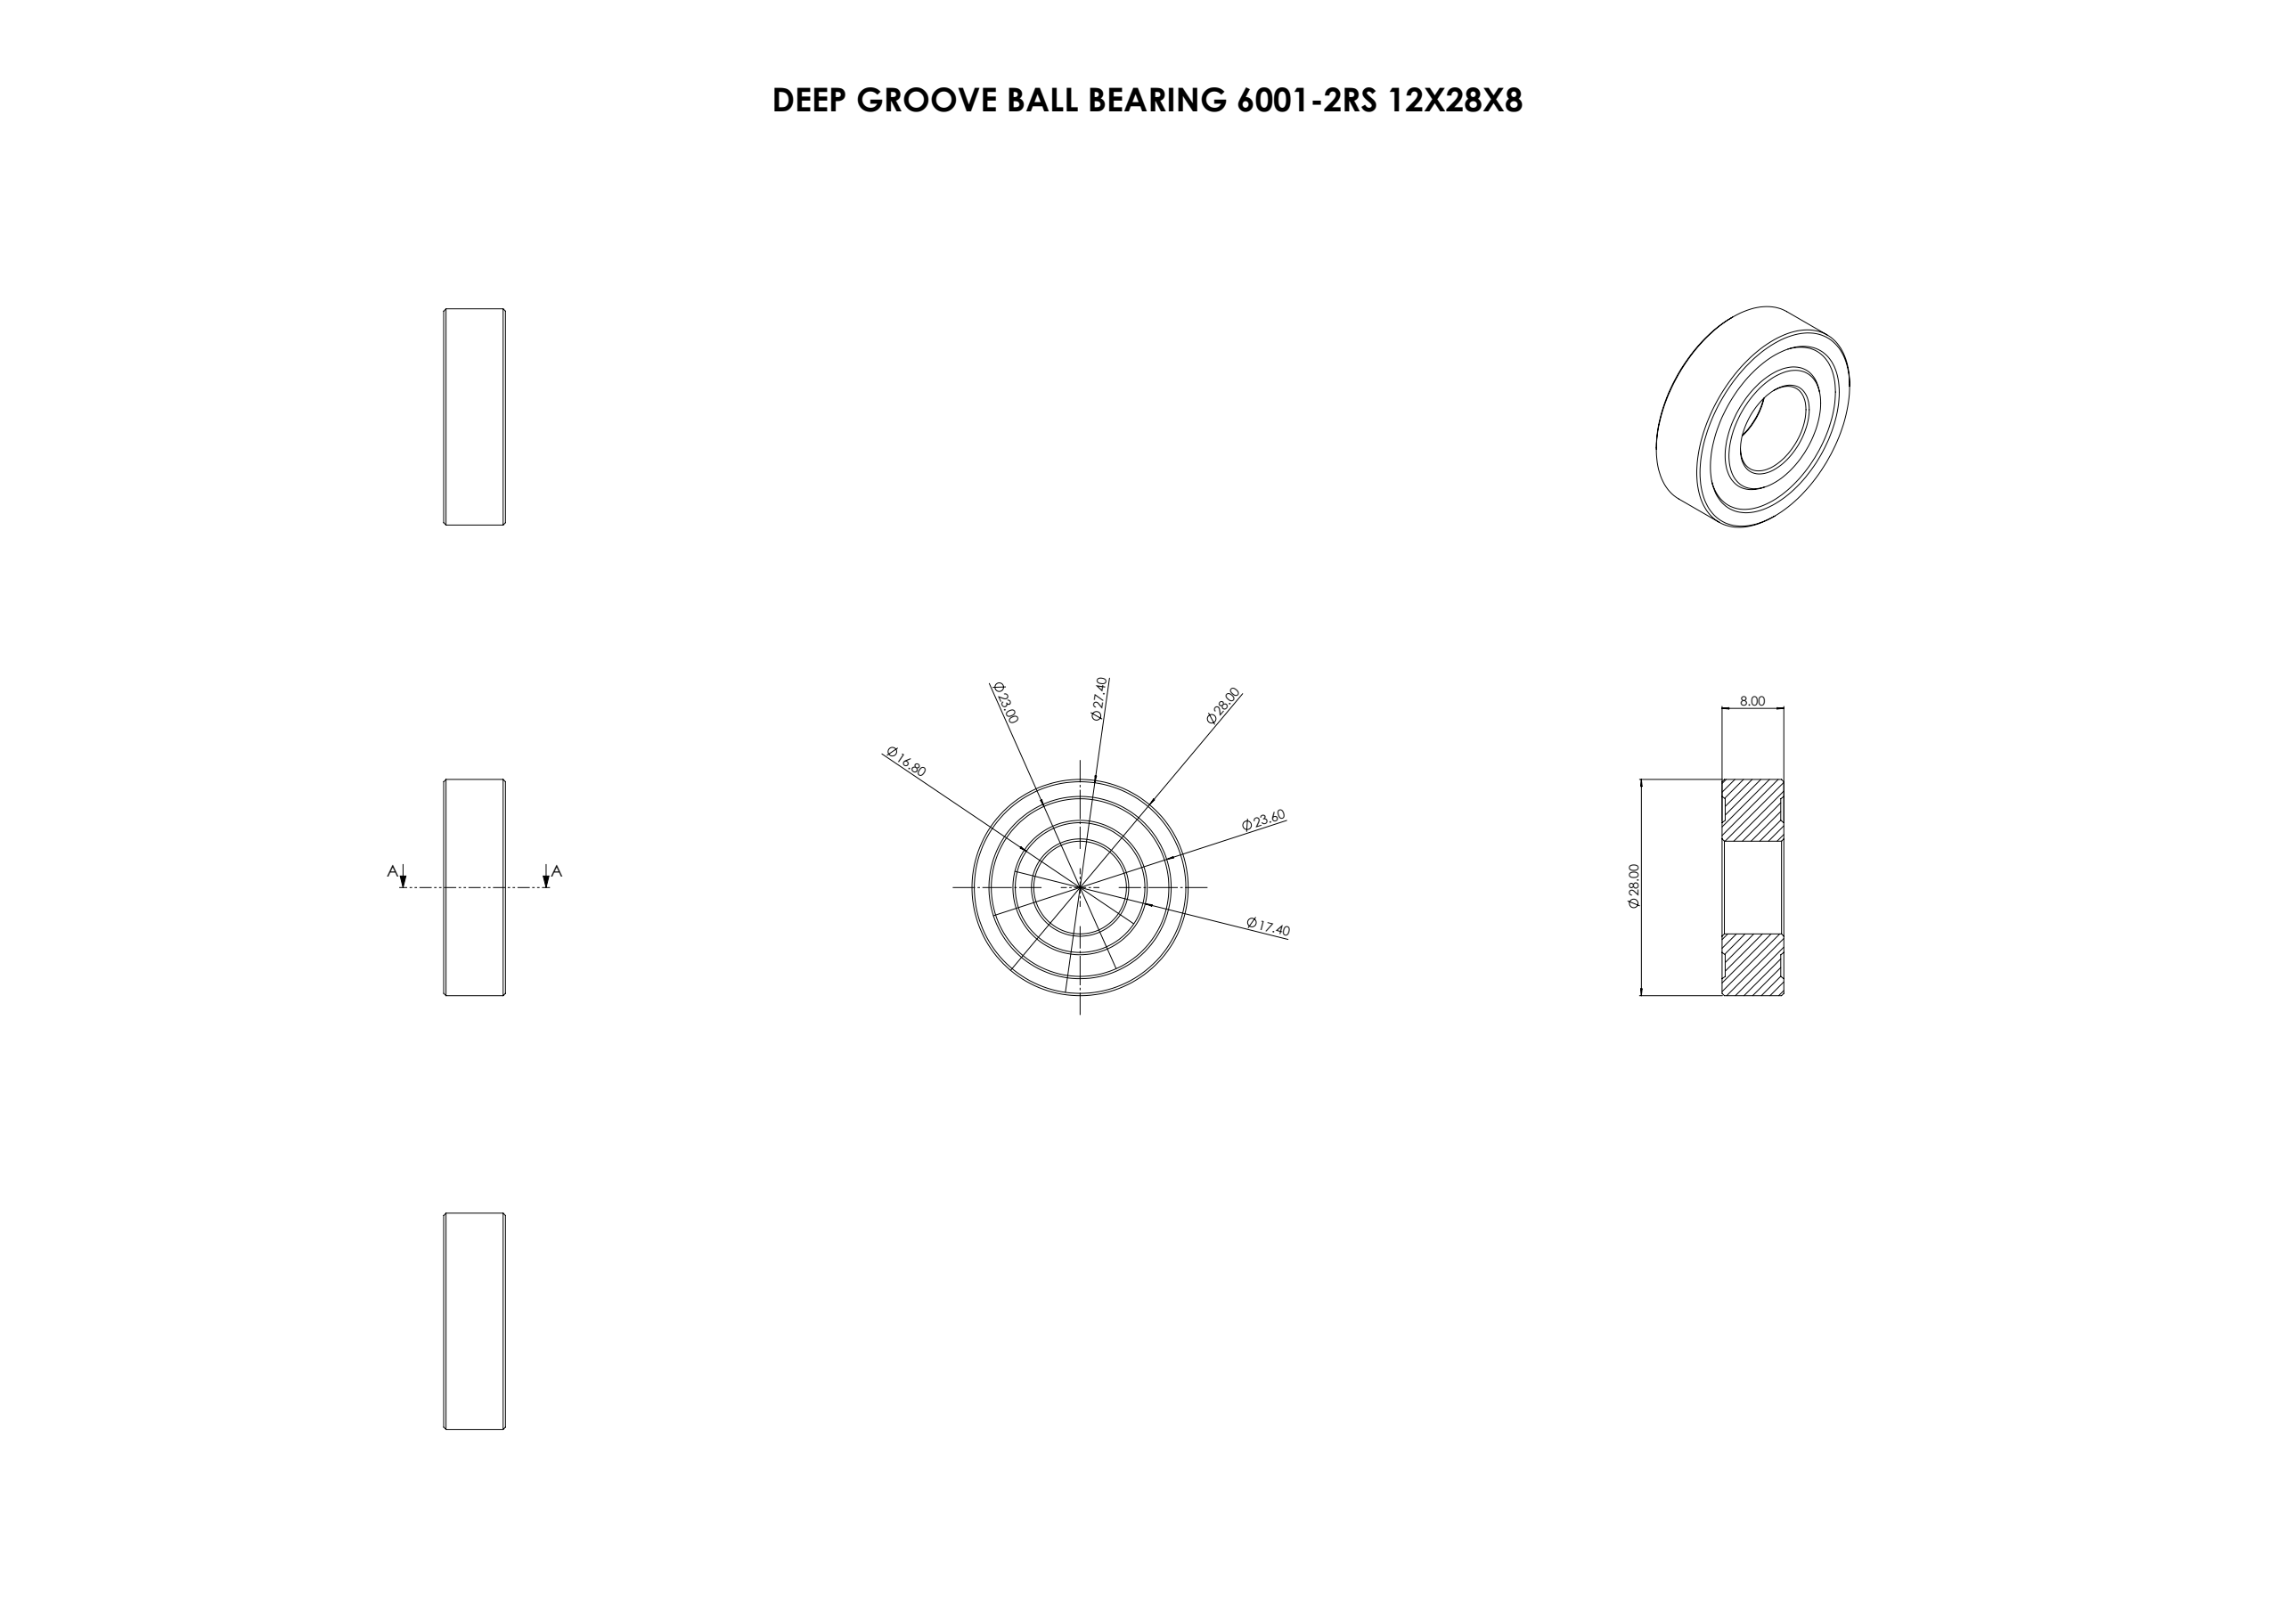
ISO-10303-21;
HEADER;
/* Generated by software containing ST-Developer
 * from STEP Tools, Inc. (www.steptools.com) 
 */

FILE_DESCRIPTION(
/* description */ (''),
/* implementation_level */ '2;1');

FILE_NAME(
/* name */ '07_Deep_Groove_Ball_Bearing_6001-2RS_12x28x8.step',
/* time_stamp */ '2026-10-11T09:12:28-07:00',
/* author */ (''),
/* organization */ (''),
/* preprocessor_version */ 'ST-DEVELOPER v20.2',
/* originating_system */ 'Autodesk Translation Framework v15.15.0.0',
/* authorisation */ '');

FILE_SCHEMA (('AUTOMOTIVE_DESIGN { 1 0 10303 214 3 1 1 }'));
ENDSEC;

DATA;
#10=MECHANICAL_DESIGN_GEOMETRIC_PRESENTATION_REPRESENTATION('',(#653),#23254);
#633=SHAPE_REPRESENTATION_RELATIONSHIP('SRR','None',#23306,#643);
#643=ADVANCED_BREP_SHAPE_REPRESENTATION('',(#663),#23250);
#653=STYLED_ITEM('',(#23462),#663);
#663=MANIFOLD_SOLID_BREP('Body1',#7031);
#748=CONICAL_SURFACE('',#7717,8.55,0.643501108793281);
#749=CONICAL_SURFACE('',#7721,11.65,0.643501108793288);
#750=CONICAL_SURFACE('',#7725,13.85,0.785398163397449);
#751=CONICAL_SURFACE('',#7729,13.85,0.785398163397448);
#752=CONICAL_SURFACE('',#7733,11.65,0.643501108793288);
#753=CONICAL_SURFACE('',#7737,8.55,0.643501108793281);
#754=CONICAL_SURFACE('',#7741,6.15,0.785398163397448);
#755=CONICAL_SURFACE('',#7745,6.15,0.785398163397449);
#838=FACE_BOUND('',#1769,.T.);
#839=FACE_BOUND('',#1772,.T.);
#840=FACE_BOUND('',#1775,.T.);
#841=FACE_BOUND('',#1780,.T.);
#842=FACE_BOUND('',#1783,.T.);
#843=FACE_BOUND('',#1786,.T.);
#952=PLANE('',#7714);
#953=PLANE('',#7719);
#954=PLANE('',#7723);
#955=PLANE('',#7731);
#956=PLANE('',#7735);
#957=PLANE('',#7739);
#1315=FACE_OUTER_BOUND('',#1768,.T.);
#1316=FACE_OUTER_BOUND('',#1770,.T.);
#1317=FACE_OUTER_BOUND('',#1771,.T.);
#1318=FACE_OUTER_BOUND('',#1773,.T.);
#1319=FACE_OUTER_BOUND('',#1774,.T.);
#1320=FACE_OUTER_BOUND('',#1776,.T.);
#1321=FACE_OUTER_BOUND('',#1777,.T.);
#1322=FACE_OUTER_BOUND('',#1778,.T.);
#1323=FACE_OUTER_BOUND('',#1779,.T.);
#1324=FACE_OUTER_BOUND('',#1781,.T.);
#1325=FACE_OUTER_BOUND('',#1782,.T.);
#1326=FACE_OUTER_BOUND('',#1784,.T.);
#1327=FACE_OUTER_BOUND('',#1785,.T.);
#1328=FACE_OUTER_BOUND('',#1787,.T.);
#1329=FACE_OUTER_BOUND('',#1788,.T.);
#1330=FACE_OUTER_BOUND('',#1789,.T.);
#1768=EDGE_LOOP('',(#6309));
#1769=EDGE_LOOP('',(#6310));
#1770=EDGE_LOOP('',(#6311,#6312,#6313,#6314));
#1771=EDGE_LOOP('',(#6315));
#1772=EDGE_LOOP('',(#6316));
#1773=EDGE_LOOP('',(#6317,#6318,#6319,#6320));
#1774=EDGE_LOOP('',(#6321));
#1775=EDGE_LOOP('',(#6322));
#1776=EDGE_LOOP('',(#6323,#6324,#6325,#6326));
#1777=EDGE_LOOP('',(#6327,#6328,#6329,#6330));
#1778=EDGE_LOOP('',(#6331,#6332,#6333,#6334));
#1779=EDGE_LOOP('',(#6335));
#1780=EDGE_LOOP('',(#6336));
#1781=EDGE_LOOP('',(#6337,#6338,#6339,#6340));
#1782=EDGE_LOOP('',(#6341));
#1783=EDGE_LOOP('',(#6342));
#1784=EDGE_LOOP('',(#6343,#6344,#6345,#6346));
#1785=EDGE_LOOP('',(#6347));
#1786=EDGE_LOOP('',(#6348));
#1787=EDGE_LOOP('',(#6349,#6350,#6351,#6352));
#1788=EDGE_LOOP('',(#6353,#6354,#6355,#6356));
#1789=EDGE_LOOP('',(#6357,#6358,#6359,#6360));
#2036=LINE('',#22022,#2295);
#2037=LINE('',#22028,#2296);
#2038=LINE('',#22036,#2297);
#2039=LINE('',#22040,#2298);
#2040=LINE('',#22044,#2299);
#2041=LINE('',#22050,#2300);
#2042=LINE('',#22058,#2301);
#2043=LINE('',#22064,#2302);
#2044=LINE('',#22068,#2303);
#2045=LINE('',#22071,#2304);
#2295=VECTOR('',#9172,8.55);
#2296=VECTOR('',#9179,11.65);
#2297=VECTOR('',#9190,13.85);
#2298=VECTOR('',#9195,14.);
#2299=VECTOR('',#9200,13.85);
#2300=VECTOR('',#9207,11.65);
#2301=VECTOR('',#9218,8.55);
#2302=VECTOR('',#9225,6.15);
#2303=VECTOR('',#9230,6.);
#2304=VECTOR('',#9235,6.15);
#2663=CIRCLE('',#7715,8.4);
#2664=CIRCLE('',#7716,6.3);
#2665=CIRCLE('',#7718,8.7);
#2666=CIRCLE('',#7720,11.5);
#2667=CIRCLE('',#7722,11.8);
#2668=CIRCLE('',#7724,13.7);
#2669=CIRCLE('',#7726,14.);
#2670=CIRCLE('',#7728,14.);
#2671=CIRCLE('',#7730,13.7);
#2672=CIRCLE('',#7732,11.8);
#2673=CIRCLE('',#7734,11.5);
#2674=CIRCLE('',#7736,8.7);
#2675=CIRCLE('',#7738,8.4);
#2676=CIRCLE('',#7740,6.3);
#2677=CIRCLE('',#7742,6.);
#2678=CIRCLE('',#7744,6.);
#3321=VERTEX_POINT('',#22015);
#3322=VERTEX_POINT('',#22017);
#3323=VERTEX_POINT('',#22020);
#3324=VERTEX_POINT('',#22024);
#3325=VERTEX_POINT('',#22027);
#3326=VERTEX_POINT('',#22031);
#3327=VERTEX_POINT('',#22034);
#3328=VERTEX_POINT('',#22038);
#3329=VERTEX_POINT('',#22042);
#3330=VERTEX_POINT('',#22046);
#3331=VERTEX_POINT('',#22049);
#3332=VERTEX_POINT('',#22053);
#3333=VERTEX_POINT('',#22056);
#3334=VERTEX_POINT('',#22060);
#3335=VERTEX_POINT('',#22063);
#3336=VERTEX_POINT('',#22067);
#4330=EDGE_CURVE('',#3321,#3321,#2663,.T.);
#4331=EDGE_CURVE('',#3322,#3322,#2664,.T.);
#4332=EDGE_CURVE('',#3323,#3323,#2665,.T.);
#4333=EDGE_CURVE('',#3323,#3321,#2036,.T.);
#4334=EDGE_CURVE('',#3324,#3324,#2666,.T.);
#4335=EDGE_CURVE('',#3324,#3325,#2037,.T.);
#4336=EDGE_CURVE('',#3325,#3325,#2667,.T.);
#4337=EDGE_CURVE('',#3326,#3326,#2668,.T.);
#4338=EDGE_CURVE('',#3327,#3327,#2669,.T.);
#4339=EDGE_CURVE('',#3327,#3326,#2038,.T.);
#4340=EDGE_CURVE('',#3328,#3328,#2670,.T.);
#4341=EDGE_CURVE('',#3328,#3327,#2039,.T.);
#4342=EDGE_CURVE('',#3329,#3329,#2671,.T.);
#4343=EDGE_CURVE('',#3329,#3328,#2040,.T.);
#4344=EDGE_CURVE('',#3330,#3330,#2672,.T.);
#4345=EDGE_CURVE('',#3330,#3331,#2041,.T.);
#4346=EDGE_CURVE('',#3331,#3331,#2673,.T.);
#4347=EDGE_CURVE('',#3332,#3332,#2674,.T.);
#4348=EDGE_CURVE('',#3333,#3333,#2675,.T.);
#4349=EDGE_CURVE('',#3333,#3332,#2042,.T.);
#4350=EDGE_CURVE('',#3334,#3334,#2676,.T.);
#4351=EDGE_CURVE('',#3334,#3335,#2043,.T.);
#4352=EDGE_CURVE('',#3335,#3335,#2677,.T.);
#4353=EDGE_CURVE('',#3335,#3336,#2044,.T.);
#4354=EDGE_CURVE('',#3336,#3336,#2678,.T.);
#4355=EDGE_CURVE('',#3336,#3322,#2045,.T.);
#6309=ORIENTED_EDGE('',*,*,#4330,.F.);
#6310=ORIENTED_EDGE('',*,*,#4331,.T.);
#6311=ORIENTED_EDGE('',*,*,#4332,.F.);
#6312=ORIENTED_EDGE('',*,*,#4333,.T.);
#6313=ORIENTED_EDGE('',*,*,#4330,.T.);
#6314=ORIENTED_EDGE('',*,*,#4333,.F.);
#6315=ORIENTED_EDGE('',*,*,#4334,.F.);
#6316=ORIENTED_EDGE('',*,*,#4332,.T.);
#6317=ORIENTED_EDGE('',*,*,#4334,.T.);
#6318=ORIENTED_EDGE('',*,*,#4335,.T.);
#6319=ORIENTED_EDGE('',*,*,#4336,.F.);
#6320=ORIENTED_EDGE('',*,*,#4335,.F.);
#6321=ORIENTED_EDGE('',*,*,#4337,.F.);
#6322=ORIENTED_EDGE('',*,*,#4336,.T.);
#6323=ORIENTED_EDGE('',*,*,#4338,.F.);
#6324=ORIENTED_EDGE('',*,*,#4339,.T.);
#6325=ORIENTED_EDGE('',*,*,#4337,.T.);
#6326=ORIENTED_EDGE('',*,*,#4339,.F.);
#6327=ORIENTED_EDGE('',*,*,#4340,.F.);
#6328=ORIENTED_EDGE('',*,*,#4341,.T.);
#6329=ORIENTED_EDGE('',*,*,#4338,.T.);
#6330=ORIENTED_EDGE('',*,*,#4341,.F.);
#6331=ORIENTED_EDGE('',*,*,#4342,.F.);
#6332=ORIENTED_EDGE('',*,*,#4343,.T.);
#6333=ORIENTED_EDGE('',*,*,#4340,.T.);
#6334=ORIENTED_EDGE('',*,*,#4343,.F.);
#6335=ORIENTED_EDGE('',*,*,#4342,.T.);
#6336=ORIENTED_EDGE('',*,*,#4344,.F.);
#6337=ORIENTED_EDGE('',*,*,#4344,.T.);
#6338=ORIENTED_EDGE('',*,*,#4345,.T.);
#6339=ORIENTED_EDGE('',*,*,#4346,.F.);
#6340=ORIENTED_EDGE('',*,*,#4345,.F.);
#6341=ORIENTED_EDGE('',*,*,#4346,.T.);
#6342=ORIENTED_EDGE('',*,*,#4347,.F.);
#6343=ORIENTED_EDGE('',*,*,#4348,.F.);
#6344=ORIENTED_EDGE('',*,*,#4349,.T.);
#6345=ORIENTED_EDGE('',*,*,#4347,.T.);
#6346=ORIENTED_EDGE('',*,*,#4349,.F.);
#6347=ORIENTED_EDGE('',*,*,#4348,.T.);
#6348=ORIENTED_EDGE('',*,*,#4350,.F.);
#6349=ORIENTED_EDGE('',*,*,#4350,.T.);
#6350=ORIENTED_EDGE('',*,*,#4351,.T.);
#6351=ORIENTED_EDGE('',*,*,#4352,.F.);
#6352=ORIENTED_EDGE('',*,*,#4351,.F.);
#6353=ORIENTED_EDGE('',*,*,#4352,.T.);
#6354=ORIENTED_EDGE('',*,*,#4353,.T.);
#6355=ORIENTED_EDGE('',*,*,#4354,.F.);
#6356=ORIENTED_EDGE('',*,*,#4353,.F.);
#6357=ORIENTED_EDGE('',*,*,#4354,.T.);
#6358=ORIENTED_EDGE('',*,*,#4355,.T.);
#6359=ORIENTED_EDGE('',*,*,#4331,.F.);
#6360=ORIENTED_EDGE('',*,*,#4355,.F.);
#6611=CYLINDRICAL_SURFACE('',#7727,14.);
#6612=CYLINDRICAL_SURFACE('',#7743,6.);
#6966=ADVANCED_FACE('',(#1315,#838),#952,.T.);
#6967=ADVANCED_FACE('',(#1316),#748,.T.);
#6968=ADVANCED_FACE('',(#1317,#839),#953,.T.);
#6969=ADVANCED_FACE('',(#1318),#749,.F.);
#6970=ADVANCED_FACE('',(#1319,#840),#954,.T.);
#6971=ADVANCED_FACE('',(#1320),#750,.T.);
#6972=ADVANCED_FACE('',(#1321),#6611,.T.);
#6973=ADVANCED_FACE('',(#1322),#751,.T.);
#6974=ADVANCED_FACE('',(#1323,#841),#955,.T.);
#6975=ADVANCED_FACE('',(#1324),#752,.F.);
#6976=ADVANCED_FACE('',(#1325,#842),#956,.T.);
#6977=ADVANCED_FACE('',(#1326),#753,.T.);
#6978=ADVANCED_FACE('',(#1327,#843),#957,.T.);
#6979=ADVANCED_FACE('',(#1328),#754,.F.);
#6980=ADVANCED_FACE('',(#1329),#6612,.F.);
#6981=ADVANCED_FACE('',(#1330),#755,.F.);
#7031=CLOSED_SHELL('',(#6966,#6967,#6968,#6969,#6970,#6971,#6972,#6973,
#6974,#6975,#6976,#6977,#6978,#6979,#6980,#6981));
#7713=AXIS2_PLACEMENT_3D('',#22013,#9160,#9161);
#7714=AXIS2_PLACEMENT_3D('',#22014,#9162,#9163);
#7715=AXIS2_PLACEMENT_3D('',#22016,#9164,#9165);
#7716=AXIS2_PLACEMENT_3D('',#22018,#9166,#9167);
#7717=AXIS2_PLACEMENT_3D('',#22019,#9168,#9169);
#7718=AXIS2_PLACEMENT_3D('',#22021,#9170,#9171);
#7719=AXIS2_PLACEMENT_3D('',#22023,#9173,#9174);
#7720=AXIS2_PLACEMENT_3D('',#22025,#9175,#9176);
#7721=AXIS2_PLACEMENT_3D('',#22026,#9177,#9178);
#7722=AXIS2_PLACEMENT_3D('',#22029,#9180,#9181);
#7723=AXIS2_PLACEMENT_3D('',#22030,#9182,#9183);
#7724=AXIS2_PLACEMENT_3D('',#22032,#9184,#9185);
#7725=AXIS2_PLACEMENT_3D('',#22033,#9186,#9187);
#7726=AXIS2_PLACEMENT_3D('',#22035,#9188,#9189);
#7727=AXIS2_PLACEMENT_3D('',#22037,#9191,#9192);
#7728=AXIS2_PLACEMENT_3D('',#22039,#9193,#9194);
#7729=AXIS2_PLACEMENT_3D('',#22041,#9196,#9197);
#7730=AXIS2_PLACEMENT_3D('',#22043,#9198,#9199);
#7731=AXIS2_PLACEMENT_3D('',#22045,#9201,#9202);
#7732=AXIS2_PLACEMENT_3D('',#22047,#9203,#9204);
#7733=AXIS2_PLACEMENT_3D('',#22048,#9205,#9206);
#7734=AXIS2_PLACEMENT_3D('',#22051,#9208,#9209);
#7735=AXIS2_PLACEMENT_3D('',#22052,#9210,#9211);
#7736=AXIS2_PLACEMENT_3D('',#22054,#9212,#9213);
#7737=AXIS2_PLACEMENT_3D('',#22055,#9214,#9215);
#7738=AXIS2_PLACEMENT_3D('',#22057,#9216,#9217);
#7739=AXIS2_PLACEMENT_3D('',#22059,#9219,#9220);
#7740=AXIS2_PLACEMENT_3D('',#22061,#9221,#9222);
#7741=AXIS2_PLACEMENT_3D('',#22062,#9223,#9224);
#7742=AXIS2_PLACEMENT_3D('',#22065,#9226,#9227);
#7743=AXIS2_PLACEMENT_3D('',#22066,#9228,#9229);
#7744=AXIS2_PLACEMENT_3D('',#22069,#9231,#9232);
#7745=AXIS2_PLACEMENT_3D('',#22070,#9233,#9234);
#9160=DIRECTION('axis',(0.,0.,1.));
#9161=DIRECTION('refdir',(1.,0.,0.));
#9162=DIRECTION('center_axis',(-1.,0.,0.));
#9163=DIRECTION('ref_axis',(0.,0.,1.));
#9164=DIRECTION('center_axis',(1.,0.,0.));
#9165=DIRECTION('ref_axis',(0.,0.,-1.));
#9166=DIRECTION('center_axis',(1.,0.,0.));
#9167=DIRECTION('ref_axis',(0.,0.,-1.));
#9168=DIRECTION('center_axis',(1.,0.,0.));
#9169=DIRECTION('ref_axis',(0.,1.,0.));
#9170=DIRECTION('center_axis',(1.,0.,0.));
#9171=DIRECTION('ref_axis',(0.,0.,-1.));
#9172=DIRECTION('',(-0.800000000000002,0.599999999999998,7.34788079488409E-17));
#9173=DIRECTION('center_axis',(-1.,0.,0.));
#9174=DIRECTION('ref_axis',(0.,0.,1.));
#9175=DIRECTION('center_axis',(1.,0.,0.));
#9176=DIRECTION('ref_axis',(0.,0.,-1.));
#9177=DIRECTION('center_axis',(-1.,0.,0.));
#9178=DIRECTION('ref_axis',(0.,1.,0.));
#9179=DIRECTION('',(-0.799999999999997,-0.600000000000003,-7.34788079488416E-17));
#9180=DIRECTION('center_axis',(1.,0.,0.));
#9181=DIRECTION('ref_axis',(0.,0.,-1.));
#9182=DIRECTION('center_axis',(-1.,0.,0.));
#9183=DIRECTION('ref_axis',(0.,0.,1.));
#9184=DIRECTION('center_axis',(1.,0.,0.));
#9185=DIRECTION('ref_axis',(0.,0.,-1.));
#9186=DIRECTION('center_axis',(1.,0.,0.));
#9187=DIRECTION('ref_axis',(0.,1.,0.));
#9188=DIRECTION('center_axis',(1.,0.,0.));
#9189=DIRECTION('ref_axis',(0.,0.,-1.));
#9190=DIRECTION('',(-0.707106781186547,0.707106781186548,8.65956056235494E-17));
#9191=DIRECTION('center_axis',(1.,0.,0.));
#9192=DIRECTION('ref_axis',(0.,1.,0.));
#9193=DIRECTION('center_axis',(1.,0.,0.));
#9194=DIRECTION('ref_axis',(0.,0.,-1.));
#9195=DIRECTION('',(-1.,0.,0.));
#9196=DIRECTION('center_axis',(-1.,0.,0.));
#9197=DIRECTION('ref_axis',(0.,1.,0.));
#9198=DIRECTION('center_axis',(1.,0.,0.));
#9199=DIRECTION('ref_axis',(0.,0.,-1.));
#9200=DIRECTION('',(-0.707106781186548,-0.707106781186548,-8.65956056235493E-17));
#9201=DIRECTION('center_axis',(1.,0.,0.));
#9202=DIRECTION('ref_axis',(0.,0.,-1.));
#9203=DIRECTION('center_axis',(1.,0.,0.));
#9204=DIRECTION('ref_axis',(0.,0.,-1.));
#9205=DIRECTION('center_axis',(1.,0.,0.));
#9206=DIRECTION('ref_axis',(0.,1.,0.));
#9207=DIRECTION('',(-0.799999999999998,0.600000000000003,7.34788079488415E-17));
#9208=DIRECTION('center_axis',(1.,0.,0.));
#9209=DIRECTION('ref_axis',(0.,0.,-1.));
#9210=DIRECTION('center_axis',(1.,0.,0.));
#9211=DIRECTION('ref_axis',(0.,0.,-1.));
#9212=DIRECTION('center_axis',(1.,0.,0.));
#9213=DIRECTION('ref_axis',(0.,0.,-1.));
#9214=DIRECTION('center_axis',(-1.,0.,0.));
#9215=DIRECTION('ref_axis',(0.,1.,0.));
#9216=DIRECTION('center_axis',(1.,0.,0.));
#9217=DIRECTION('ref_axis',(0.,0.,-1.));
#9218=DIRECTION('',(-0.800000000000002,-0.599999999999997,-7.34788079488409E-17));
#9219=DIRECTION('center_axis',(1.,0.,0.));
#9220=DIRECTION('ref_axis',(0.,0.,-1.));
#9221=DIRECTION('center_axis',(1.,0.,0.));
#9222=DIRECTION('ref_axis',(0.,0.,-1.));
#9223=DIRECTION('center_axis',(1.,0.,0.));
#9224=DIRECTION('ref_axis',(0.,1.,0.));
#9225=DIRECTION('',(-0.707106781186548,0.707106781186548,8.65956056235493E-17));
#9226=DIRECTION('center_axis',(1.,0.,0.));
#9227=DIRECTION('ref_axis',(0.,0.,-1.));
#9228=DIRECTION('center_axis',(1.,0.,0.));
#9229=DIRECTION('ref_axis',(0.,1.,0.));
#9230=DIRECTION('',(-1.,0.,0.));
#9231=DIRECTION('center_axis',(1.,0.,0.));
#9232=DIRECTION('ref_axis',(0.,0.,-1.));
#9233=DIRECTION('center_axis',(-1.,0.,0.));
#9234=DIRECTION('ref_axis',(0.,1.,0.));
#9235=DIRECTION('',(-0.707106781186547,-0.707106781186548,-8.65956056235494E-17));
#22013=CARTESIAN_POINT('',(0.,0.,0.));
#22014=CARTESIAN_POINT('Origin',(0.,8.4,0.));
#22015=CARTESIAN_POINT('',(-3.12250225675825E-16,-8.4,-1.02870331128378E-15));
#22016=CARTESIAN_POINT('Origin',(0.,0.,0.));
#22017=CARTESIAN_POINT('',(-6.93889390390723E-17,-6.3,-7.71527483462833E-16));
#22018=CARTESIAN_POINT('Origin',(0.,0.,0.));
#22019=CARTESIAN_POINT('Origin',(0.2,0.,0.));
#22020=CARTESIAN_POINT('',(0.4,-8.7,-1.0654427152582E-15));
#22021=CARTESIAN_POINT('Origin',(0.4,0.,0.));
#22022=CARTESIAN_POINT('',(0.2,-8.55,-1.04707301327099E-15));
#22023=CARTESIAN_POINT('Origin',(0.4,11.5,0.));
#22024=CARTESIAN_POINT('',(0.4,-11.5,-1.40834381901946E-15));
#22025=CARTESIAN_POINT('Origin',(0.4,0.,0.));
#22026=CARTESIAN_POINT('Origin',(0.2,0.,0.));
#22027=CARTESIAN_POINT('',(-4.5102810375397E-16,-11.8,-1.44508322299388E-15));
#22028=CARTESIAN_POINT('',(0.2,-11.65,-1.42671352100667E-15));
#22029=CARTESIAN_POINT('Origin',(0.,0.,0.));
#22030=CARTESIAN_POINT('Origin',(0.,13.7,0.));
#22031=CARTESIAN_POINT('',(2.94902990916057E-16,-13.7,-1.67776611483187E-15));
#22032=CARTESIAN_POINT('Origin',(0.,0.,0.));
#22033=CARTESIAN_POINT('Origin',(0.15,0.,0.));
#22034=CARTESIAN_POINT('',(0.300000000000001,-14.,-1.71450551880629E-15));
#22035=CARTESIAN_POINT('Origin',(0.3,0.,0.));
#22036=CARTESIAN_POINT('',(0.15,-13.85,-1.69613581681908E-15));
#22037=CARTESIAN_POINT('Origin',(4.,0.,0.));
#22038=CARTESIAN_POINT('',(7.7,-14.,-1.71450551880629E-15));
#22039=CARTESIAN_POINT('Origin',(7.7,0.,0.));
#22040=CARTESIAN_POINT('',(4.,-14.,-1.71450551880629E-15));
#22041=CARTESIAN_POINT('Origin',(7.85,0.,0.));
#22042=CARTESIAN_POINT('',(8.,-13.7,-1.67776611483187E-15));
#22043=CARTESIAN_POINT('Origin',(8.,0.,0.));
#22044=CARTESIAN_POINT('',(7.85,-13.85,-1.69613581681908E-15));
#22045=CARTESIAN_POINT('Origin',(8.,11.8,0.));
#22046=CARTESIAN_POINT('',(8.,-11.8,-1.44508322299388E-15));
#22047=CARTESIAN_POINT('Origin',(8.,0.,0.));
#22048=CARTESIAN_POINT('Origin',(7.8,0.,0.));
#22049=CARTESIAN_POINT('',(7.6,-11.5,-1.40834381901946E-15));
#22050=CARTESIAN_POINT('',(7.8,-11.65,-1.42671352100667E-15));
#22051=CARTESIAN_POINT('Origin',(7.6,0.,0.));
#22052=CARTESIAN_POINT('Origin',(7.6,8.7,0.));
#22053=CARTESIAN_POINT('',(7.6,-8.7,-1.0654427152582E-15));
#22054=CARTESIAN_POINT('Origin',(7.6,0.,0.));
#22055=CARTESIAN_POINT('Origin',(7.8,0.,0.));
#22056=CARTESIAN_POINT('',(8.,-8.4,-1.02870331128378E-15));
#22057=CARTESIAN_POINT('Origin',(8.,0.,0.));
#22058=CARTESIAN_POINT('',(7.8,-8.55,-1.04707301327099E-15));
#22059=CARTESIAN_POINT('Origin',(8.,6.3,0.));
#22060=CARTESIAN_POINT('',(8.,-6.3,-7.71527483462833E-16));
#22061=CARTESIAN_POINT('Origin',(8.,0.,0.));
#22062=CARTESIAN_POINT('Origin',(7.85,0.,0.));
#22063=CARTESIAN_POINT('',(7.7,-6.,-7.34788079488412E-16));
#22064=CARTESIAN_POINT('',(7.85,-6.15,-7.53157781475622E-16));
#22065=CARTESIAN_POINT('Origin',(7.7,0.,0.));
#22066=CARTESIAN_POINT('Origin',(4.,0.,0.));
#22067=CARTESIAN_POINT('',(0.3,-6.,-7.34788079488412E-16));
#22068=CARTESIAN_POINT('',(4.,-6.,-7.34788079488412E-16));
#22069=CARTESIAN_POINT('Origin',(0.3,0.,0.));
#22070=CARTESIAN_POINT('Origin',(0.15,0.,0.));
#22071=CARTESIAN_POINT('',(0.15,-6.15,-7.53157781475622E-16));
#23238=UNCERTAINTY_MEASURE_WITH_UNIT(LENGTH_MEASURE(0.01),#23255,
'DISTANCE_ACCURACY_VALUE',
'Maximum model space distance between geometric entities at asserted c
onnectivities');
#23242=UNCERTAINTY_MEASURE_WITH_UNIT(LENGTH_MEASURE(0.01),#23255,
'DISTANCE_ACCURACY_VALUE',
'Maximum model space distance between geometric entities at asserted c
onnectivities');
#23250=(
GEOMETRIC_REPRESENTATION_CONTEXT(3)
GLOBAL_UNCERTAINTY_ASSIGNED_CONTEXT((#23238))
GLOBAL_UNIT_ASSIGNED_CONTEXT((#23255,#23257,#23258))
REPRESENTATION_CONTEXT('','3D')
);
#23254=(
GEOMETRIC_REPRESENTATION_CONTEXT(3)
GLOBAL_UNCERTAINTY_ASSIGNED_CONTEXT((#23242))
GLOBAL_UNIT_ASSIGNED_CONTEXT((#23255,#23257,#23258))
REPRESENTATION_CONTEXT('','3D')
);
#23255=(
LENGTH_UNIT()
NAMED_UNIT(*)
SI_UNIT(.MILLI.,.METRE.)
);
#23257=(
NAMED_UNIT(*)
PLANE_ANGLE_UNIT()
SI_UNIT($,.RADIAN.)
);
#23258=(
NAMED_UNIT(*)
SI_UNIT($,.STERADIAN.)
SOLID_ANGLE_UNIT()
);
#23266=SHAPE_DEFINITION_REPRESENTATION(#23277,#23306);
#23277=PRODUCT_DEFINITION_SHAPE('',$,#23318);
#23306=SHAPE_REPRESENTATION('',(#7713),#23250);
#23310=PRODUCT_DEFINITION_CONTEXT('part definition',#23345,'design');
#23318=PRODUCT_DEFINITION('2026-10-11-09-11-54-369',
'07_Deep_Groove_Ball_Bearing_6001-2RS_12x28x8',#23329,#23310);
#23329=PRODUCT_DEFINITION_FORMATION('',$,#23354);
#23345=APPLICATION_CONTEXT(
'Core Data for Automotive Mechanical Design Process');
#23346=PRODUCT_CONTEXT('part definition',#23345,'mechanical');
#23354=PRODUCT('2026-10-11-09-11-54-369',
'07_Deep_Groove_Ball_Bearing_6001-2RS_12x28x8',$,(#23346));
#23456=COLOUR_RGB('Grey',0.48,0.52,0.57);
#23457=FILL_AREA_STYLE_COLOUR('',#23456);
#23458=FILL_AREA_STYLE('',(#23457));
#23459=SURFACE_STYLE_FILL_AREA(#23458);
#23460=SURFACE_SIDE_STYLE('',(#23459));
#23461=SURFACE_STYLE_USAGE(.BOTH.,#23460);
#23462=PRESENTATION_STYLE_ASSIGNMENT((#23461));
ENDSEC;
END-ISO-10303-21;
